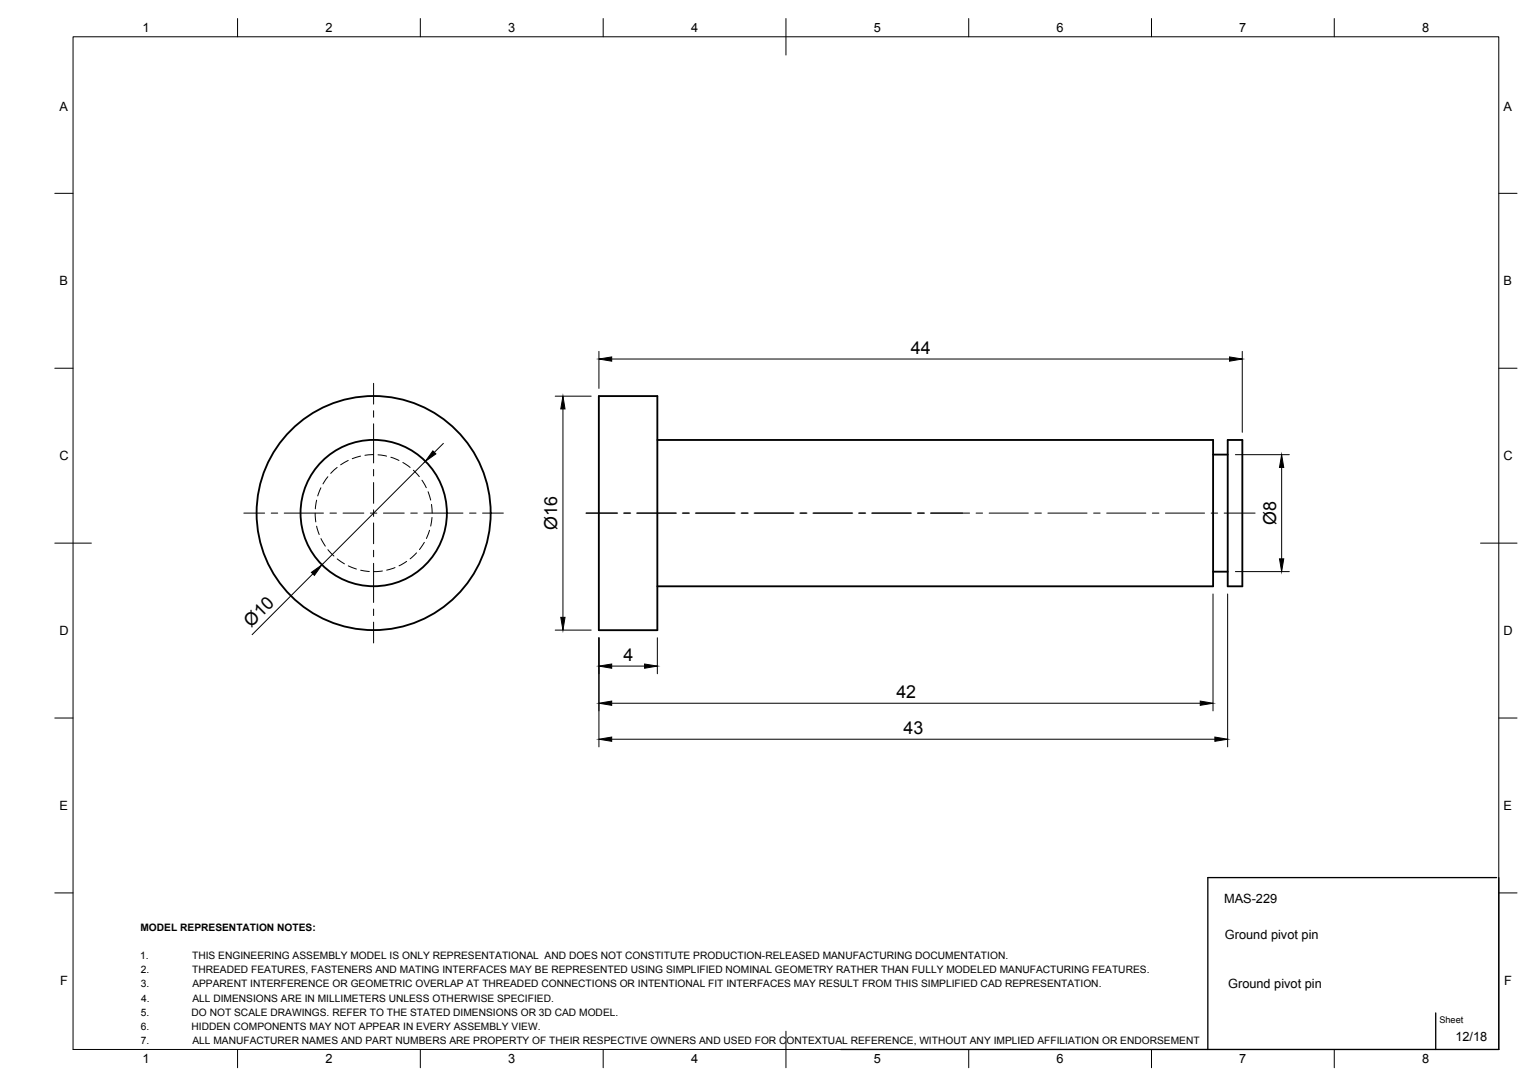
ISO-10303-21;
HEADER;
/* Generated by software containing ST-Developer
 * from STEP Tools, Inc. (www.steptools.com) 
 */

FILE_DESCRIPTION(
/* description */ ('Independently dimensioned six-bar single-leg walking-linkage demonstr
ator. Whole-mm20 crank,60 upper rocker,80/120 ternary coupler,120 lowe
r rocker,140 knee pitch and260 toe reach; ground pivots0/0,60/0,40/60.
 Seven native revolutes close both loops. Four reused native library f
amilies, fully retained shared pins and layered real spacer stacks, bo
nded rubber toe. Benchtop reference mechanism; no complete vehicle, lo
ad, gait stability, adhesive, weld, fit or life rating.'),
/* implementation_level */ '2;1');

FILE_NAME(
/* name */ 'Ground pivot pin.step',
/* time_stamp */ '2026-11-09T20:33:14-08:00',
/* author */ (''),
/* organization */ (''),
/* preprocessor_version */ 'ST-DEVELOPER v20.2',
/* originating_system */ 'Autodesk Translation Framework v15.17.0.0',
/* authorisation */ '');

FILE_SCHEMA (('AUTOMOTIVE_DESIGN { 1 0 10303 214 3 1 1 }'));
ENDSEC;

DATA;
#10=MECHANICAL_DESIGN_GEOMETRIC_PRESENTATION_REPRESENTATION('',(#264),#4048);
#228=SHAPE_REPRESENTATION_RELATIONSHIP('SRR','None',#4152,#246);
#246=ADVANCED_BREP_SHAPE_REPRESENTATION('',(#282),#4039);
#264=STYLED_ITEM('',(#4251),#282);
#282=MANIFOLD_SOLID_BREP('Body1',#2153);
#329=FACE_BOUND('',#650,.T.);
#330=FACE_BOUND('',#652,.T.);
#331=FACE_BOUND('',#655,.T.);
#386=PLANE('',#2506);
#387=PLANE('',#2508);
#388=PLANE('',#2512);
#389=PLANE('',#2517);
#390=PLANE('',#2519);
#484=FACE_OUTER_BOUND('',#648,.T.);
#485=FACE_OUTER_BOUND('',#649,.T.);
#486=FACE_OUTER_BOUND('',#651,.T.);
#487=FACE_OUTER_BOUND('',#653,.T.);
#488=FACE_OUTER_BOUND('',#654,.T.);
#489=FACE_OUTER_BOUND('',#656,.T.);
#490=FACE_OUTER_BOUND('',#657,.T.);
#491=FACE_OUTER_BOUND('',#658,.T.);
#492=FACE_OUTER_BOUND('',#659,.T.);
#648=EDGE_LOOP('',(#1791,#1792,#1793,#1794));
#649=EDGE_LOOP('',(#1795));
#650=EDGE_LOOP('',(#1796));
#651=EDGE_LOOP('',(#1797));
#652=EDGE_LOOP('',(#1798));
#653=EDGE_LOOP('',(#1799,#1800,#1801,#1802));
#654=EDGE_LOOP('',(#1803));
#655=EDGE_LOOP('',(#1804));
#656=EDGE_LOOP('',(#1805,#1806,#1807,#1808));
#657=EDGE_LOOP('',(#1809));
#658=EDGE_LOOP('',(#1810,#1811,#1812,#1813));
#659=EDGE_LOOP('',(#1814));
#815=LINE('',#3755,#940);
#816=LINE('',#3766,#941);
#817=LINE('',#3774,#942);
#818=LINE('',#3778,#943);
#940=VECTOR('',#3050,4.);
#941=VECTOR('',#3065,5.);
#942=VECTOR('',#3074,8.);
#943=VECTOR('',#3081,5.);
#1036=CIRCLE('',#2504,4.);
#1037=CIRCLE('',#2505,4.);
#1038=CIRCLE('',#2507,5.);
#1039=CIRCLE('',#2509,5.);
#1040=CIRCLE('',#2511,5.);
#1041=CIRCLE('',#2513,8.);
#1042=CIRCLE('',#2514,5.);
#1043=CIRCLE('',#2516,8.);
#1190=VERTEX_POINT('',#3752);
#1191=VERTEX_POINT('',#3754);
#1192=VERTEX_POINT('',#3758);
#1193=VERTEX_POINT('',#3761);
#1194=VERTEX_POINT('',#3764);
#1195=VERTEX_POINT('',#3768);
#1196=VERTEX_POINT('',#3770);
#1197=VERTEX_POINT('',#3773);
#1399=EDGE_CURVE('',#1190,#1190,#1036,.T.);
#1400=EDGE_CURVE('',#1190,#1191,#815,.T.);
#1401=EDGE_CURVE('',#1191,#1191,#1037,.T.);
#1402=EDGE_CURVE('',#1192,#1192,#1038,.T.);
#1403=EDGE_CURVE('',#1193,#1193,#1039,.T.);
#1404=EDGE_CURVE('',#1194,#1194,#1040,.T.);
#1405=EDGE_CURVE('',#1194,#1193,#816,.T.);
#1406=EDGE_CURVE('',#1195,#1195,#1041,.T.);
#1407=EDGE_CURVE('',#1196,#1196,#1042,.T.);
#1408=EDGE_CURVE('',#1195,#1197,#817,.T.);
#1409=EDGE_CURVE('',#1197,#1197,#1043,.T.);
#1410=EDGE_CURVE('',#1192,#1196,#818,.T.);
#1791=ORIENTED_EDGE('',*,*,#1399,.T.);
#1792=ORIENTED_EDGE('',*,*,#1400,.T.);
#1793=ORIENTED_EDGE('',*,*,#1401,.F.);
#1794=ORIENTED_EDGE('',*,*,#1400,.F.);
#1795=ORIENTED_EDGE('',*,*,#1402,.F.);
#1796=ORIENTED_EDGE('',*,*,#1399,.F.);
#1797=ORIENTED_EDGE('',*,*,#1403,.F.);
#1798=ORIENTED_EDGE('',*,*,#1401,.T.);
#1799=ORIENTED_EDGE('',*,*,#1404,.F.);
#1800=ORIENTED_EDGE('',*,*,#1405,.T.);
#1801=ORIENTED_EDGE('',*,*,#1403,.T.);
#1802=ORIENTED_EDGE('',*,*,#1405,.F.);
#1803=ORIENTED_EDGE('',*,*,#1406,.T.);
#1804=ORIENTED_EDGE('',*,*,#1407,.F.);
#1805=ORIENTED_EDGE('',*,*,#1406,.F.);
#1806=ORIENTED_EDGE('',*,*,#1408,.T.);
#1807=ORIENTED_EDGE('',*,*,#1409,.T.);
#1808=ORIENTED_EDGE('',*,*,#1408,.F.);
#1809=ORIENTED_EDGE('',*,*,#1409,.F.);
#1810=ORIENTED_EDGE('',*,*,#1402,.T.);
#1811=ORIENTED_EDGE('',*,*,#1410,.T.);
#1812=ORIENTED_EDGE('',*,*,#1407,.T.);
#1813=ORIENTED_EDGE('',*,*,#1410,.F.);
#1814=ORIENTED_EDGE('',*,*,#1404,.T.);
#1994=CYLINDRICAL_SURFACE('',#2503,4.);
#1995=CYLINDRICAL_SURFACE('',#2510,5.);
#1996=CYLINDRICAL_SURFACE('',#2515,8.);
#1997=CYLINDRICAL_SURFACE('',#2518,5.);
#2087=ADVANCED_FACE('',(#484),#1994,.T.);
#2088=ADVANCED_FACE('',(#485,#329),#386,.F.);
#2089=ADVANCED_FACE('',(#486,#330),#387,.F.);
#2090=ADVANCED_FACE('',(#487),#1995,.T.);
#2091=ADVANCED_FACE('',(#488,#331),#388,.T.);
#2092=ADVANCED_FACE('',(#489),#1996,.T.);
#2093=ADVANCED_FACE('',(#490),#389,.F.);
#2094=ADVANCED_FACE('',(#491),#1997,.T.);
#2095=ADVANCED_FACE('',(#492),#390,.T.);
#2153=CLOSED_SHELL('',(#2087,#2088,#2089,#2090,#2091,#2092,#2093,#2094,
#2095));
#2502=AXIS2_PLACEMENT_3D('',#3750,#3044,#3045);
#2503=AXIS2_PLACEMENT_3D('',#3751,#3046,#3047);
#2504=AXIS2_PLACEMENT_3D('',#3753,#3048,#3049);
#2505=AXIS2_PLACEMENT_3D('',#3756,#3051,#3052);
#2506=AXIS2_PLACEMENT_3D('',#3757,#3053,#3054);
#2507=AXIS2_PLACEMENT_3D('',#3759,#3055,#3056);
#2508=AXIS2_PLACEMENT_3D('',#3760,#3057,#3058);
#2509=AXIS2_PLACEMENT_3D('',#3762,#3059,#3060);
#2510=AXIS2_PLACEMENT_3D('',#3763,#3061,#3062);
#2511=AXIS2_PLACEMENT_3D('',#3765,#3063,#3064);
#2512=AXIS2_PLACEMENT_3D('',#3767,#3066,#3067);
#2513=AXIS2_PLACEMENT_3D('',#3769,#3068,#3069);
#2514=AXIS2_PLACEMENT_3D('',#3771,#3070,#3071);
#2515=AXIS2_PLACEMENT_3D('',#3772,#3072,#3073);
#2516=AXIS2_PLACEMENT_3D('',#3775,#3075,#3076);
#2517=AXIS2_PLACEMENT_3D('',#3776,#3077,#3078);
#2518=AXIS2_PLACEMENT_3D('',#3777,#3079,#3080);
#2519=AXIS2_PLACEMENT_3D('',#3779,#3082,#3083);
#3044=DIRECTION('axis',(0.,0.,1.));
#3045=DIRECTION('refdir',(1.,0.,0.));
#3046=DIRECTION('center_axis',(0.,0.,1.));
#3047=DIRECTION('ref_axis',(1.,0.,0.));
#3048=DIRECTION('center_axis',(0.,0.,1.));
#3049=DIRECTION('ref_axis',(1.,0.,0.));
#3050=DIRECTION('',(0.,0.,1.));
#3051=DIRECTION('center_axis',(0.,0.,1.));
#3052=DIRECTION('ref_axis',(1.,0.,0.));
#3053=DIRECTION('center_axis',(0.,0.,-1.));
#3054=DIRECTION('ref_axis',(-1.,0.,0.));
#3055=DIRECTION('center_axis',(0.,0.,-1.));
#3056=DIRECTION('ref_axis',(1.,0.,0.));
#3057=DIRECTION('center_axis',(0.,0.,1.));
#3058=DIRECTION('ref_axis',(1.,0.,0.));
#3059=DIRECTION('center_axis',(0.,0.,1.));
#3060=DIRECTION('ref_axis',(1.,0.,0.));
#3061=DIRECTION('center_axis',(0.,0.,1.));
#3062=DIRECTION('ref_axis',(1.,0.,0.));
#3063=DIRECTION('center_axis',(0.,0.,1.));
#3064=DIRECTION('ref_axis',(1.,0.,0.));
#3065=DIRECTION('',(0.,0.,-1.));
#3066=DIRECTION('center_axis',(0.,0.,1.));
#3067=DIRECTION('ref_axis',(1.,0.,0.));
#3068=DIRECTION('center_axis',(0.,0.,1.));
#3069=DIRECTION('ref_axis',(1.,0.,0.));
#3070=DIRECTION('center_axis',(0.,0.,1.));
#3071=DIRECTION('ref_axis',(1.,0.,0.));
#3072=DIRECTION('center_axis',(0.,0.,1.));
#3073=DIRECTION('ref_axis',(1.,0.,0.));
#3074=DIRECTION('',(0.,0.,-1.));
#3075=DIRECTION('center_axis',(0.,0.,1.));
#3076=DIRECTION('ref_axis',(1.,0.,0.));
#3077=DIRECTION('center_axis',(0.,0.,1.));
#3078=DIRECTION('ref_axis',(1.,0.,0.));
#3079=DIRECTION('center_axis',(0.,0.,1.));
#3080=DIRECTION('ref_axis',(1.,0.,0.));
#3081=DIRECTION('',(0.,0.,-1.));
#3082=DIRECTION('center_axis',(0.,0.,1.));
#3083=DIRECTION('ref_axis',(1.,0.,0.));
#3750=CARTESIAN_POINT('',(0.,0.,0.));
#3751=CARTESIAN_POINT('Origin',(0.,0.,38.5));
#3752=CARTESIAN_POINT('',(-4.,-4.89858719658941E-16,38.));
#3753=CARTESIAN_POINT('Origin',(0.,0.,38.));
#3754=CARTESIAN_POINT('',(-4.,-4.89858719658941E-16,39.));
#3755=CARTESIAN_POINT('',(-4.,-4.89858719658941E-16,38.5));
#3756=CARTESIAN_POINT('Origin',(0.,0.,39.));
#3757=CARTESIAN_POINT('Origin',(8.,0.,38.));
#3758=CARTESIAN_POINT('',(-5.,6.12323399573677E-16,38.));
#3759=CARTESIAN_POINT('Origin',(0.,0.,38.));
#3760=CARTESIAN_POINT('Origin',(4.,0.,39.));
#3761=CARTESIAN_POINT('',(-5.,-6.12323399573677E-16,39.));
#3762=CARTESIAN_POINT('Origin',(0.,0.,39.));
#3763=CARTESIAN_POINT('Origin',(0.,0.,0.));
#3764=CARTESIAN_POINT('',(-5.,-6.12323399573677E-16,40.));
#3765=CARTESIAN_POINT('Origin',(0.,0.,40.));
#3766=CARTESIAN_POINT('',(-5.,-6.12323399573677E-16,0.));
#3767=CARTESIAN_POINT('Origin',(0.,0.,0.));
#3768=CARTESIAN_POINT('',(-8.,-9.79717439317883E-16,0.));
#3769=CARTESIAN_POINT('Origin',(0.,0.,0.));
#3770=CARTESIAN_POINT('',(-5.,-6.12323399573677E-16,0.));
#3771=CARTESIAN_POINT('Origin',(0.,0.,0.));
#3772=CARTESIAN_POINT('Origin',(0.,0.,-4.));
#3773=CARTESIAN_POINT('',(-8.,-9.79717439317883E-16,-4.));
#3774=CARTESIAN_POINT('',(-8.,-9.79717439317883E-16,-4.));
#3775=CARTESIAN_POINT('Origin',(0.,0.,-4.));
#3776=CARTESIAN_POINT('Origin',(0.,0.,-4.));
#3777=CARTESIAN_POINT('Origin',(0.,0.,0.));
#3778=CARTESIAN_POINT('',(-5.,-6.12323399573677E-16,0.));
#3779=CARTESIAN_POINT('Origin',(0.,0.,40.));
#4019=UNCERTAINTY_MEASURE_WITH_UNIT(LENGTH_MEASURE(0.01),#4049,
'DISTANCE_ACCURACY_VALUE',
'Maximum model space distance between geometric entities at asserted c
onnectivities');
#4028=UNCERTAINTY_MEASURE_WITH_UNIT(LENGTH_MEASURE(0.01),#4049,
'DISTANCE_ACCURACY_VALUE',
'Maximum model space distance between geometric entities at asserted c
onnectivities');
#4039=(
GEOMETRIC_REPRESENTATION_CONTEXT(3)
GLOBAL_UNCERTAINTY_ASSIGNED_CONTEXT((#4019))
GLOBAL_UNIT_ASSIGNED_CONTEXT((#4049,#4051,#4052))
REPRESENTATION_CONTEXT('','3D')
);
#4048=(
GEOMETRIC_REPRESENTATION_CONTEXT(3)
GLOBAL_UNCERTAINTY_ASSIGNED_CONTEXT((#4028))
GLOBAL_UNIT_ASSIGNED_CONTEXT((#4049,#4051,#4052))
REPRESENTATION_CONTEXT('','3D')
);
#4049=(
LENGTH_UNIT()
NAMED_UNIT(*)
SI_UNIT(.MILLI.,.METRE.)
);
#4051=(
NAMED_UNIT(*)
PLANE_ANGLE_UNIT()
SI_UNIT($,.RADIAN.)
);
#4052=(
NAMED_UNIT(*)
SI_UNIT($,.STERADIAN.)
SOLID_ANGLE_UNIT()
);
#4063=SHAPE_DEFINITION_REPRESENTATION(#4082,#4152);
#4082=PRODUCT_DEFINITION_SHAPE('',$,#4172);
#4152=SHAPE_REPRESENTATION('',(#2502),#4039);
#4161=PRODUCT_DEFINITION_CONTEXT('part definition',#4220,'design');
#4172=PRODUCT_DEFINITION('Ground pivot pin','Ground pivot pin',#4191,#4161);
#4191=PRODUCT_DEFINITION_FORMATION('',$,#4232);
#4220=APPLICATION_CONTEXT(
'Core Data for Automotive Mechanical Design Process');
#4221=PRODUCT_CONTEXT('part definition',#4220,'mechanical');
#4232=PRODUCT('Ground pivot pin','Ground pivot pin',$,(#4221));
#4251=PRESENTATION_STYLE_ASSIGNMENT((#4265));
#4265=SURFACE_STYLE_USAGE(.BOTH.,#4279);
#4279=SURFACE_SIDE_STYLE('',(#4293));
#4293=SURFACE_STYLE_FILL_AREA(#4307);
#4307=FILL_AREA_STYLE('Pin gray',(#4321));
#4321=FILL_AREA_STYLE_COLOUR('Pin gray',#4335);
#4335=COLOUR_RGB('Pin gray',0.576470588235294,0.615686274509804,0.666666666666667);
ENDSEC;
END-ISO-10303-21;
